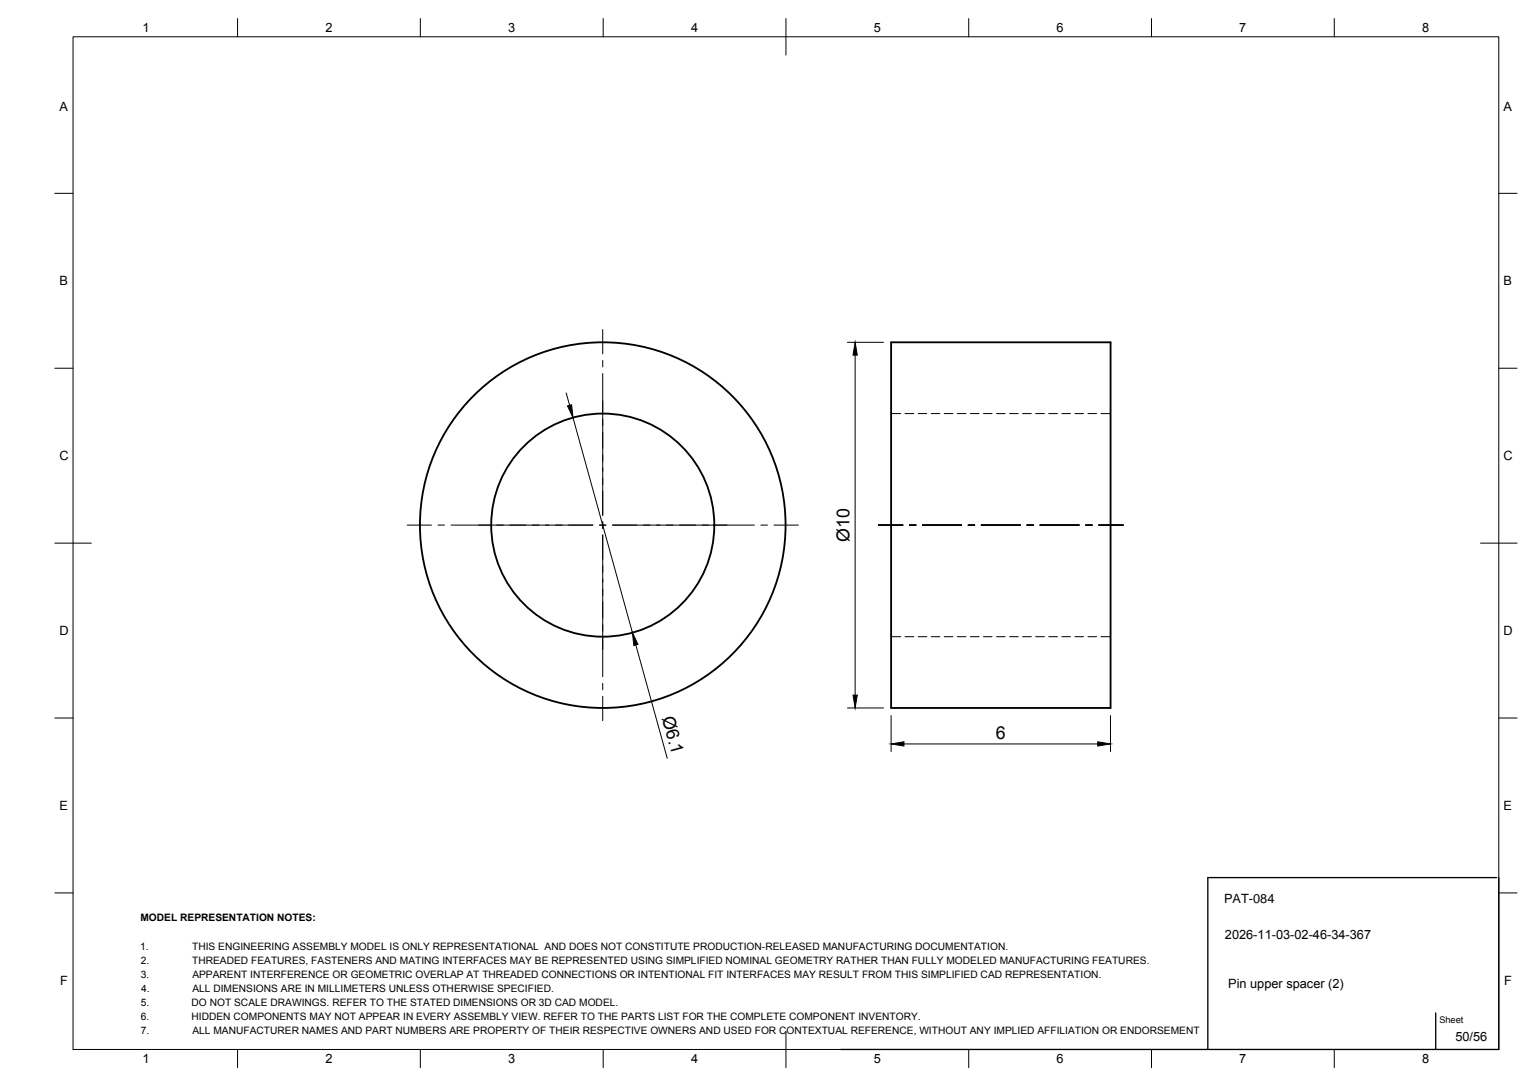
ISO-10303-21;
HEADER;
/* Generated by software containing ST-Developer
 * from STEP Tools, Inc. (www.steptools.com) 
 */

FILE_DESCRIPTION(
/* description */ ('Quick-return (Whitworth) mechanism'),
/* implementation_level */ '2;1');

FILE_NAME(
/* name */ 'Pin upper spacer (2).step',
/* time_stamp */ '2026-10-28T03:25:57-07:00',
/* author */ (''),
/* organization */ (''),
/* preprocessor_version */ 'ST-DEVELOPER v20.2',
/* originating_system */ 'Autodesk Translation Framework v15.17.0.0',
/* authorisation */ '');

FILE_SCHEMA (('AUTOMOTIVE_DESIGN { 1 0 10303 214 3 1 1 }'));
ENDSEC;

DATA;
#10=MECHANICAL_DESIGN_GEOMETRIC_PRESENTATION_REPRESENTATION('',(#535),#14878);
#439=SHAPE_REPRESENTATION_RELATIONSHIP('SRR','None',#15113,#483);
#483=ADVANCED_BREP_SHAPE_REPRESENTATION('',(#586),#14870);
#535=STYLED_ITEM('',(#15406),#586);
#586=MANIFOLD_SOLID_BREP('Body1',#7890);
#772=FACE_BOUND('',#2081,.T.);
#773=FACE_BOUND('',#2083,.T.);
#983=PLANE('',#9206);
#984=PLANE('',#9207);
#1431=FACE_OUTER_BOUND('',#2078,.T.);
#1432=FACE_OUTER_BOUND('',#2079,.T.);
#1433=FACE_OUTER_BOUND('',#2080,.T.);
#1434=FACE_OUTER_BOUND('',#2082,.T.);
#2078=EDGE_LOOP('',(#6826,#6827,#6828,#6829));
#2079=EDGE_LOOP('',(#6830,#6831,#6832,#6833));
#2080=EDGE_LOOP('',(#6834));
#2081=EDGE_LOOP('',(#6835));
#2082=EDGE_LOOP('',(#6836));
#2083=EDGE_LOOP('',(#6837));
#2539=LINE('',#14298,#3062);
#2540=LINE('',#14304,#3063);
#3062=VECTOR('',#11402,0.305);
#3063=VECTOR('',#11409,0.5);
#3593=CIRCLE('',#9201,0.305);
#3594=CIRCLE('',#9202,0.305);
#3595=CIRCLE('',#9204,0.5);
#3596=CIRCLE('',#9205,0.5);
#4162=VERTEX_POINT('',#14295);
#4163=VERTEX_POINT('',#14297);
#4164=VERTEX_POINT('',#14301);
#4165=VERTEX_POINT('',#14303);
#5070=EDGE_CURVE('',#4162,#4162,#3593,.T.);
#5071=EDGE_CURVE('',#4162,#4163,#2539,.T.);
#5072=EDGE_CURVE('',#4163,#4163,#3594,.T.);
#5073=EDGE_CURVE('',#4164,#4164,#3595,.T.);
#5074=EDGE_CURVE('',#4164,#4165,#2540,.T.);
#5075=EDGE_CURVE('',#4165,#4165,#3596,.T.);
#6826=ORIENTED_EDGE('',*,*,#5070,.F.);
#6827=ORIENTED_EDGE('',*,*,#5071,.T.);
#6828=ORIENTED_EDGE('',*,*,#5072,.T.);
#6829=ORIENTED_EDGE('',*,*,#5071,.F.);
#6830=ORIENTED_EDGE('',*,*,#5073,.F.);
#6831=ORIENTED_EDGE('',*,*,#5074,.T.);
#6832=ORIENTED_EDGE('',*,*,#5075,.T.);
#6833=ORIENTED_EDGE('',*,*,#5074,.F.);
#6834=ORIENTED_EDGE('',*,*,#5073,.T.);
#6835=ORIENTED_EDGE('',*,*,#5070,.T.);
#6836=ORIENTED_EDGE('',*,*,#5075,.F.);
#6837=ORIENTED_EDGE('',*,*,#5072,.F.);
#7366=CYLINDRICAL_SURFACE('',#9200,0.305);
#7367=CYLINDRICAL_SURFACE('',#9203,0.5);
#7762=ADVANCED_FACE('',(#1431),#7366,.F.);
#7763=ADVANCED_FACE('',(#1432),#7367,.T.);
#7764=ADVANCED_FACE('',(#1433,#772),#983,.T.);
#7765=ADVANCED_FACE('',(#1434,#773),#984,.F.);
#7890=CLOSED_SHELL('',(#7762,#7763,#7764,#7765));
#9199=AXIS2_PLACEMENT_3D('',#14293,#11396,#11397);
#9200=AXIS2_PLACEMENT_3D('',#14294,#11398,#11399);
#9201=AXIS2_PLACEMENT_3D('',#14296,#11400,#11401);
#9202=AXIS2_PLACEMENT_3D('',#14299,#11403,#11404);
#9203=AXIS2_PLACEMENT_3D('',#14300,#11405,#11406);
#9204=AXIS2_PLACEMENT_3D('',#14302,#11407,#11408);
#9205=AXIS2_PLACEMENT_3D('',#14305,#11410,#11411);
#9206=AXIS2_PLACEMENT_3D('',#14306,#11412,#11413);
#9207=AXIS2_PLACEMENT_3D('',#14307,#11414,#11415);
#11396=DIRECTION('axis',(0.,0.,1.));
#11397=DIRECTION('refdir',(1.,0.,0.));
#11398=DIRECTION('center_axis',(0.,0.,1.));
#11399=DIRECTION('ref_axis',(1.,0.,0.));
#11400=DIRECTION('center_axis',(0.,0.,-1.));
#11401=DIRECTION('ref_axis',(1.,0.,0.));
#11402=DIRECTION('',(0.,0.,-1.));
#11403=DIRECTION('center_axis',(0.,0.,-1.));
#11404=DIRECTION('ref_axis',(1.,0.,0.));
#11405=DIRECTION('center_axis',(0.,0.,1.));
#11406=DIRECTION('ref_axis',(1.,0.,0.));
#11407=DIRECTION('center_axis',(0.,0.,1.));
#11408=DIRECTION('ref_axis',(1.,0.,0.));
#11409=DIRECTION('',(0.,0.,-1.));
#11410=DIRECTION('center_axis',(0.,0.,1.));
#11411=DIRECTION('ref_axis',(1.,0.,0.));
#11412=DIRECTION('center_axis',(0.,0.,1.));
#11413=DIRECTION('ref_axis',(1.,0.,0.));
#11414=DIRECTION('center_axis',(0.,0.,1.));
#11415=DIRECTION('ref_axis',(1.,0.,0.));
#14293=CARTESIAN_POINT('',(0.,0.,0.));
#14294=CARTESIAN_POINT('Origin',(9.16515138991168,16.,9.2));
#14295=CARTESIAN_POINT('',(8.86015138991168,16.,9.8));
#14296=CARTESIAN_POINT('Origin',(9.16515138991168,16.,9.8));
#14297=CARTESIAN_POINT('',(8.86015138991168,16.,9.2));
#14298=CARTESIAN_POINT('',(8.86015138991168,16.,9.2));
#14299=CARTESIAN_POINT('Origin',(9.16515138991168,16.,9.2));
#14300=CARTESIAN_POINT('Origin',(9.16515138991168,16.,9.2));
#14301=CARTESIAN_POINT('',(8.66515138991168,16.,9.8));
#14302=CARTESIAN_POINT('Origin',(9.16515138991168,16.,9.8));
#14303=CARTESIAN_POINT('',(8.66515138991168,16.,9.2));
#14304=CARTESIAN_POINT('',(8.66515138991168,16.,9.2));
#14305=CARTESIAN_POINT('Origin',(9.16515138991168,16.,9.2));
#14306=CARTESIAN_POINT('Origin',(9.16515138991168,16.,9.8));
#14307=CARTESIAN_POINT('Origin',(9.16515138991168,16.,9.2));
#14816=UNCERTAINTY_MEASURE_WITH_UNIT(LENGTH_MEASURE(0.001),#14879,
'DISTANCE_ACCURACY_VALUE',
'Maximum model space distance between geometric entities at asserted c
onnectivities');
#14824=UNCERTAINTY_MEASURE_WITH_UNIT(LENGTH_MEASURE(0.001),#14879,
'DISTANCE_ACCURACY_VALUE',
'Maximum model space distance between geometric entities at asserted c
onnectivities');
#14870=(
GEOMETRIC_REPRESENTATION_CONTEXT(3)
GLOBAL_UNCERTAINTY_ASSIGNED_CONTEXT((#14816))
GLOBAL_UNIT_ASSIGNED_CONTEXT((#14879,#14881,#14882))
REPRESENTATION_CONTEXT('','3D')
);
#14878=(
GEOMETRIC_REPRESENTATION_CONTEXT(3)
GLOBAL_UNCERTAINTY_ASSIGNED_CONTEXT((#14824))
GLOBAL_UNIT_ASSIGNED_CONTEXT((#14879,#14881,#14882))
REPRESENTATION_CONTEXT('','3D')
);
#14879=(
LENGTH_UNIT()
NAMED_UNIT(*)
SI_UNIT(.CENTI.,.METRE.)
);
#14881=(
NAMED_UNIT(*)
PLANE_ANGLE_UNIT()
SI_UNIT($,.RADIAN.)
);
#14882=(
NAMED_UNIT(*)
SI_UNIT($,.STERADIAN.)
SOLID_ANGLE_UNIT()
);
#14928=SHAPE_DEFINITION_REPRESENTATION(#14990,#15113);
#14990=PRODUCT_DEFINITION_SHAPE('',$,#15167);
#15113=SHAPE_REPRESENTATION('',(#9199),#14870);
#15121=PRODUCT_DEFINITION_CONTEXT('part definition',#15282,'design');
#15167=PRODUCT_DEFINITION('Pin upper spacer (2)','Pin upper spacer (2)',#15220,
#15121);
#15220=PRODUCT_DEFINITION_FORMATION('',$,#15329);
#15282=APPLICATION_CONTEXT(
'Core Data for Automotive Mechanical Design Process');
#15283=PRODUCT_CONTEXT('part definition',#15282,'mechanical');
#15329=PRODUCT('Pin upper spacer (2)','Pin upper spacer (2)',
'Pin upper spacer (2)',(#15283));
#15400=COLOUR_RGB('Grey',0.48,0.52,0.57);
#15401=FILL_AREA_STYLE_COLOUR('',#15400);
#15402=FILL_AREA_STYLE('',(#15401));
#15403=SURFACE_STYLE_FILL_AREA(#15402);
#15404=SURFACE_SIDE_STYLE('',(#15403));
#15405=SURFACE_STYLE_USAGE(.BOTH.,#15404);
#15406=PRESENTATION_STYLE_ASSIGNMENT((#15405));
ENDSEC;
END-ISO-10303-21;
